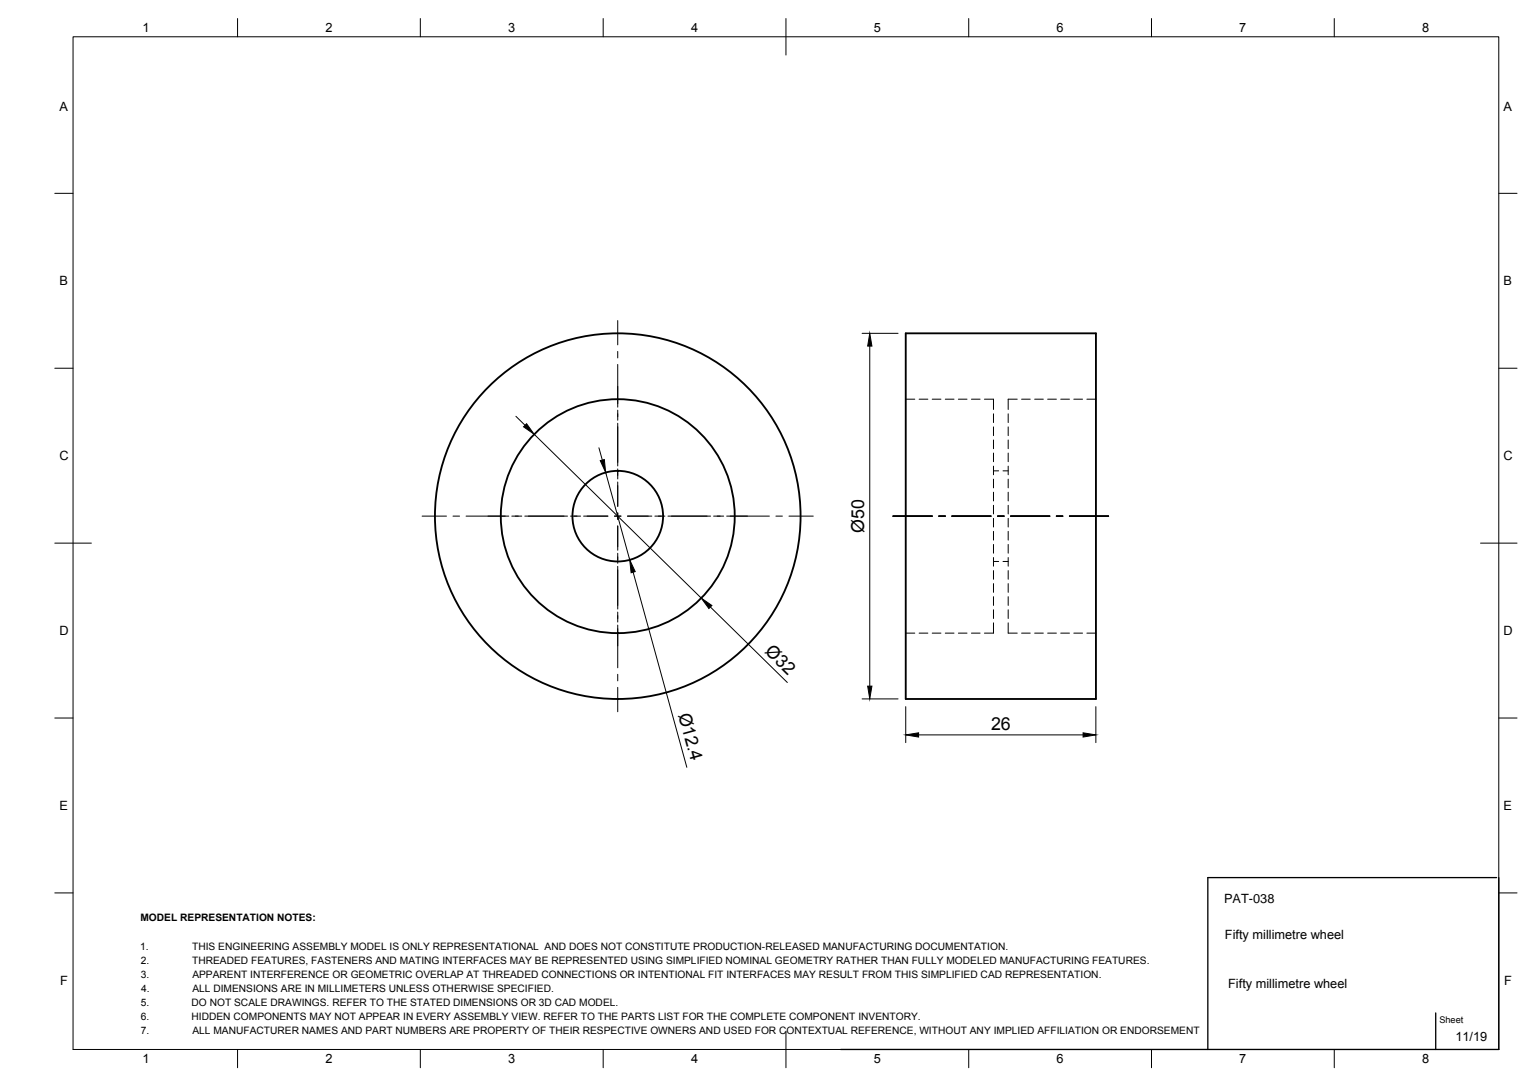
ISO-10303-21;
HEADER;
/* Generated by software containing ST-Developer
 * from STEP Tools, Inc. (www.steptools.com) 
 */

FILE_DESCRIPTION(
/* description */ ('Fork-mounted skate wheel'),
/* implementation_level */ '2;1');

FILE_NAME(
/* name */ 'Fifty millimetre wheel.step',
/* time_stamp */ '2026-10-29T16:11:26-07:00',
/* author */ (''),
/* organization */ (''),
/* preprocessor_version */ 'ST-DEVELOPER v20.2',
/* originating_system */ 'Autodesk Translation Framework v15.17.0.0',
/* authorisation */ '');

FILE_SCHEMA (('AUTOMOTIVE_DESIGN { 1 0 10303 214 3 1 1 }'));
ENDSEC;

DATA;
#10=MECHANICAL_DESIGN_GEOMETRIC_PRESENTATION_REPRESENTATION('',(#151),#3688);
#127=SHAPE_REPRESENTATION_RELATIONSHIP('SRR','None',#3751,#139);
#139=ADVANCED_BREP_SHAPE_REPRESENTATION('',(#169),#3680);
#151=STYLED_ITEM('',(#3882),#169);
#169=MANIFOLD_SOLID_BREP('Body1',#1813);
#204=FACE_BOUND('',#465,.T.);
#205=FACE_BOUND('',#468,.T.);
#206=FACE_BOUND('',#472,.T.);
#207=FACE_BOUND('',#474,.T.);
#254=PLANE('',#2064);
#255=PLANE('',#2069);
#256=PLANE('',#2075);
#257=PLANE('',#2076);
#329=FACE_OUTER_BOUND('',#463,.T.);
#330=FACE_OUTER_BOUND('',#464,.T.);
#331=FACE_OUTER_BOUND('',#466,.T.);
#332=FACE_OUTER_BOUND('',#467,.T.);
#333=FACE_OUTER_BOUND('',#469,.T.);
#334=FACE_OUTER_BOUND('',#470,.T.);
#335=FACE_OUTER_BOUND('',#471,.T.);
#336=FACE_OUTER_BOUND('',#473,.T.);
#463=EDGE_LOOP('',(#1427,#1428,#1429,#1430));
#464=EDGE_LOOP('',(#1431));
#465=EDGE_LOOP('',(#1432));
#466=EDGE_LOOP('',(#1433,#1434,#1435,#1436));
#467=EDGE_LOOP('',(#1437));
#468=EDGE_LOOP('',(#1438));
#469=EDGE_LOOP('',(#1439,#1440,#1441,#1442));
#470=EDGE_LOOP('',(#1443,#1444,#1445,#1446));
#471=EDGE_LOOP('',(#1447));
#472=EDGE_LOOP('',(#1448));
#473=EDGE_LOOP('',(#1449));
#474=EDGE_LOOP('',(#1450));
#610=LINE('',#3083,#704);
#611=LINE('',#3092,#705);
#612=LINE('',#3098,#706);
#613=LINE('',#3103,#707);
#704=VECTOR('',#2499,1.6);
#705=VECTOR('',#2510,1.6);
#706=VECTOR('',#2519,0.62);
#707=VECTOR('',#2524,2.5);
#759=CIRCLE('',#2062,1.6);
#760=CIRCLE('',#2063,1.6);
#761=CIRCLE('',#2065,0.62);
#762=CIRCLE('',#2067,1.6);
#763=CIRCLE('',#2068,1.6);
#764=CIRCLE('',#2070,0.62);
#765=CIRCLE('',#2073,2.5);
#766=CIRCLE('',#2074,2.5);
#909=VERTEX_POINT('',#3080);
#910=VERTEX_POINT('',#3082);
#911=VERTEX_POINT('',#3086);
#912=VERTEX_POINT('',#3089);
#913=VERTEX_POINT('',#3091);
#914=VERTEX_POINT('',#3095);
#915=VERTEX_POINT('',#3100);
#916=VERTEX_POINT('',#3102);
#1100=EDGE_CURVE('',#909,#909,#759,.T.);
#1101=EDGE_CURVE('',#909,#910,#610,.T.);
#1102=EDGE_CURVE('',#910,#910,#760,.T.);
#1103=EDGE_CURVE('',#911,#911,#761,.T.);
#1104=EDGE_CURVE('',#912,#912,#762,.T.);
#1105=EDGE_CURVE('',#912,#913,#611,.T.);
#1106=EDGE_CURVE('',#913,#913,#763,.T.);
#1107=EDGE_CURVE('',#914,#914,#764,.T.);
#1108=EDGE_CURVE('',#911,#914,#612,.T.);
#1109=EDGE_CURVE('',#915,#915,#765,.T.);
#1110=EDGE_CURVE('',#915,#916,#613,.T.);
#1111=EDGE_CURVE('',#916,#916,#766,.T.);
#1427=ORIENTED_EDGE('',*,*,#1100,.F.);
#1428=ORIENTED_EDGE('',*,*,#1101,.T.);
#1429=ORIENTED_EDGE('',*,*,#1102,.F.);
#1430=ORIENTED_EDGE('',*,*,#1101,.F.);
#1431=ORIENTED_EDGE('',*,*,#1100,.T.);
#1432=ORIENTED_EDGE('',*,*,#1103,.F.);
#1433=ORIENTED_EDGE('',*,*,#1104,.F.);
#1434=ORIENTED_EDGE('',*,*,#1105,.T.);
#1435=ORIENTED_EDGE('',*,*,#1106,.T.);
#1436=ORIENTED_EDGE('',*,*,#1105,.F.);
#1437=ORIENTED_EDGE('',*,*,#1106,.F.);
#1438=ORIENTED_EDGE('',*,*,#1107,.F.);
#1439=ORIENTED_EDGE('',*,*,#1103,.T.);
#1440=ORIENTED_EDGE('',*,*,#1108,.T.);
#1441=ORIENTED_EDGE('',*,*,#1107,.T.);
#1442=ORIENTED_EDGE('',*,*,#1108,.F.);
#1443=ORIENTED_EDGE('',*,*,#1109,.F.);
#1444=ORIENTED_EDGE('',*,*,#1110,.T.);
#1445=ORIENTED_EDGE('',*,*,#1111,.T.);
#1446=ORIENTED_EDGE('',*,*,#1110,.F.);
#1447=ORIENTED_EDGE('',*,*,#1109,.T.);
#1448=ORIENTED_EDGE('',*,*,#1102,.T.);
#1449=ORIENTED_EDGE('',*,*,#1111,.F.);
#1450=ORIENTED_EDGE('',*,*,#1104,.T.);
#1676=CYLINDRICAL_SURFACE('',#2061,1.6);
#1677=CYLINDRICAL_SURFACE('',#2066,1.6);
#1678=CYLINDRICAL_SURFACE('',#2071,0.62);
#1679=CYLINDRICAL_SURFACE('',#2072,2.5);
#1747=ADVANCED_FACE('',(#329),#1676,.F.);
#1748=ADVANCED_FACE('',(#330,#204),#254,.T.);
#1749=ADVANCED_FACE('',(#331),#1677,.F.);
#1750=ADVANCED_FACE('',(#332,#205),#255,.F.);
#1751=ADVANCED_FACE('',(#333),#1678,.F.);
#1752=ADVANCED_FACE('',(#334),#1679,.T.);
#1753=ADVANCED_FACE('',(#335,#206),#256,.T.);
#1754=ADVANCED_FACE('',(#336,#207),#257,.F.);
#1813=CLOSED_SHELL('',(#1747,#1748,#1749,#1750,#1751,#1752,#1753,#1754));
#2060=AXIS2_PLACEMENT_3D('',#3078,#2493,#2494);
#2061=AXIS2_PLACEMENT_3D('',#3079,#2495,#2496);
#2062=AXIS2_PLACEMENT_3D('',#3081,#2497,#2498);
#2063=AXIS2_PLACEMENT_3D('',#3084,#2500,#2501);
#2064=AXIS2_PLACEMENT_3D('',#3085,#2502,#2503);
#2065=AXIS2_PLACEMENT_3D('',#3087,#2504,#2505);
#2066=AXIS2_PLACEMENT_3D('',#3088,#2506,#2507);
#2067=AXIS2_PLACEMENT_3D('',#3090,#2508,#2509);
#2068=AXIS2_PLACEMENT_3D('',#3093,#2511,#2512);
#2069=AXIS2_PLACEMENT_3D('',#3094,#2513,#2514);
#2070=AXIS2_PLACEMENT_3D('',#3096,#2515,#2516);
#2071=AXIS2_PLACEMENT_3D('',#3097,#2517,#2518);
#2072=AXIS2_PLACEMENT_3D('',#3099,#2520,#2521);
#2073=AXIS2_PLACEMENT_3D('',#3101,#2522,#2523);
#2074=AXIS2_PLACEMENT_3D('',#3104,#2525,#2526);
#2075=AXIS2_PLACEMENT_3D('',#3105,#2527,#2528);
#2076=AXIS2_PLACEMENT_3D('',#3106,#2529,#2530);
#2493=DIRECTION('axis',(0.,0.,1.));
#2494=DIRECTION('refdir',(1.,0.,0.));
#2495=DIRECTION('center_axis',(0.,1.,0.));
#2496=DIRECTION('ref_axis',(1.,0.,0.));
#2497=DIRECTION('center_axis',(0.,1.,0.));
#2498=DIRECTION('ref_axis',(1.,0.,0.));
#2499=DIRECTION('',(0.,1.,0.));
#2500=DIRECTION('center_axis',(0.,-1.,0.));
#2501=DIRECTION('ref_axis',(1.,0.,0.));
#2502=DIRECTION('center_axis',(0.,1.,0.));
#2503=DIRECTION('ref_axis',(1.,0.,0.));
#2504=DIRECTION('center_axis',(0.,1.,0.));
#2505=DIRECTION('ref_axis',(1.,0.,0.));
#2506=DIRECTION('center_axis',(0.,1.,0.));
#2507=DIRECTION('ref_axis',(1.,0.,0.));
#2508=DIRECTION('center_axis',(0.,1.,0.));
#2509=DIRECTION('ref_axis',(1.,0.,0.));
#2510=DIRECTION('',(0.,1.,0.));
#2511=DIRECTION('center_axis',(0.,1.,0.));
#2512=DIRECTION('ref_axis',(1.,0.,0.));
#2513=DIRECTION('center_axis',(0.,1.,0.));
#2514=DIRECTION('ref_axis',(1.,0.,0.));
#2515=DIRECTION('center_axis',(0.,-1.,0.));
#2516=DIRECTION('ref_axis',(1.,0.,0.));
#2517=DIRECTION('center_axis',(0.,1.,0.));
#2518=DIRECTION('ref_axis',(1.,0.,0.));
#2519=DIRECTION('',(0.,-1.,0.));
#2520=DIRECTION('center_axis',(0.,1.,0.));
#2521=DIRECTION('ref_axis',(1.,0.,0.));
#2522=DIRECTION('center_axis',(0.,1.,0.));
#2523=DIRECTION('ref_axis',(1.,0.,0.));
#2524=DIRECTION('',(0.,-1.,0.));
#2525=DIRECTION('center_axis',(0.,1.,0.));
#2526=DIRECTION('ref_axis',(1.,0.,0.));
#2527=DIRECTION('center_axis',(0.,1.,0.));
#2528=DIRECTION('ref_axis',(1.,0.,0.));
#2529=DIRECTION('center_axis',(0.,1.,0.));
#2530=DIRECTION('ref_axis',(1.,0.,0.));
#3078=CARTESIAN_POINT('',(0.,0.,0.));
#3079=CARTESIAN_POINT('Origin',(0.,0.1,3.5));
#3080=CARTESIAN_POINT('',(-1.6,0.1,3.5));
#3081=CARTESIAN_POINT('Origin',(0.,0.1,3.5));
#3082=CARTESIAN_POINT('',(-1.6,1.3,3.5));
#3083=CARTESIAN_POINT('',(-1.6,0.1,3.5));
#3084=CARTESIAN_POINT('Origin',(0.,1.3,3.5));
#3085=CARTESIAN_POINT('Origin',(0.,0.1,3.5));
#3086=CARTESIAN_POINT('',(-0.62,0.1,3.5));
#3087=CARTESIAN_POINT('Origin',(0.,0.1,3.5));
#3088=CARTESIAN_POINT('Origin',(0.,-1.4,3.5));
#3089=CARTESIAN_POINT('',(-1.6,-1.3,3.5));
#3090=CARTESIAN_POINT('Origin',(0.,-1.3,3.5));
#3091=CARTESIAN_POINT('',(-1.6,-0.1,3.5));
#3092=CARTESIAN_POINT('',(-1.6,-1.4,3.5));
#3093=CARTESIAN_POINT('Origin',(0.,-0.1,3.5));
#3094=CARTESIAN_POINT('Origin',(0.,-0.1,3.5));
#3095=CARTESIAN_POINT('',(-0.62,-0.1,3.5));
#3096=CARTESIAN_POINT('Origin',(0.,-0.1,3.5));
#3097=CARTESIAN_POINT('Origin',(0.,-1.3,3.5));
#3098=CARTESIAN_POINT('',(-0.62,-1.3,3.5));
#3099=CARTESIAN_POINT('Origin',(0.,-1.3,3.5));
#3100=CARTESIAN_POINT('',(-2.5,1.3,3.5));
#3101=CARTESIAN_POINT('Origin',(0.,1.3,3.5));
#3102=CARTESIAN_POINT('',(-2.5,-1.3,3.5));
#3103=CARTESIAN_POINT('',(-2.5,-1.3,3.5));
#3104=CARTESIAN_POINT('Origin',(0.,-1.3,3.5));
#3105=CARTESIAN_POINT('Origin',(0.,1.3,3.5));
#3106=CARTESIAN_POINT('Origin',(0.,-1.3,3.5));
#3663=UNCERTAINTY_MEASURE_WITH_UNIT(LENGTH_MEASURE(0.001),#3689,
'DISTANCE_ACCURACY_VALUE',
'Maximum model space distance between geometric entities at asserted c
onnectivities');
#3671=UNCERTAINTY_MEASURE_WITH_UNIT(LENGTH_MEASURE(0.001),#3689,
'DISTANCE_ACCURACY_VALUE',
'Maximum model space distance between geometric entities at asserted c
onnectivities');
#3680=(
GEOMETRIC_REPRESENTATION_CONTEXT(3)
GLOBAL_UNCERTAINTY_ASSIGNED_CONTEXT((#3663))
GLOBAL_UNIT_ASSIGNED_CONTEXT((#3689,#3691,#3692))
REPRESENTATION_CONTEXT('','3D')
);
#3688=(
GEOMETRIC_REPRESENTATION_CONTEXT(3)
GLOBAL_UNCERTAINTY_ASSIGNED_CONTEXT((#3671))
GLOBAL_UNIT_ASSIGNED_CONTEXT((#3689,#3691,#3692))
REPRESENTATION_CONTEXT('','3D')
);
#3689=(
LENGTH_UNIT()
NAMED_UNIT(*)
SI_UNIT(.CENTI.,.METRE.)
);
#3691=(
NAMED_UNIT(*)
PLANE_ANGLE_UNIT()
SI_UNIT($,.RADIAN.)
);
#3692=(
NAMED_UNIT(*)
SI_UNIT($,.STERADIAN.)
SOLID_ANGLE_UNIT()
);
#3701=SHAPE_DEFINITION_REPRESENTATION(#3723,#3751);
#3723=PRODUCT_DEFINITION_SHAPE('',$,#3768);
#3751=SHAPE_REPRESENTATION('',(#2060),#3680);
#3759=PRODUCT_DEFINITION_CONTEXT('part definition',#3809,'design');
#3768=PRODUCT_DEFINITION('Fifty millimetre wheel',
'Fifty millimetre wheel',#3784,#3759);
#3784=PRODUCT_DEFINITION_FORMATION('',$,#3819);
#3809=APPLICATION_CONTEXT(
'Core Data for Automotive Mechanical Design Process');
#3810=PRODUCT_CONTEXT('part definition',#3809,'mechanical');
#3819=PRODUCT('Fifty millimetre wheel','Fifty millimetre wheel',
'Fifty millimetre wheel',(#3810));
#3876=COLOUR_RGB('Light Blue',0.38,0.62,0.78);
#3877=FILL_AREA_STYLE_COLOUR('',#3876);
#3878=FILL_AREA_STYLE('',(#3877));
#3879=SURFACE_STYLE_FILL_AREA(#3878);
#3880=SURFACE_SIDE_STYLE('',(#3879));
#3881=SURFACE_STYLE_USAGE(.BOTH.,#3880);
#3882=PRESENTATION_STYLE_ASSIGNMENT((#3881));
ENDSEC;
END-ISO-10303-21;
